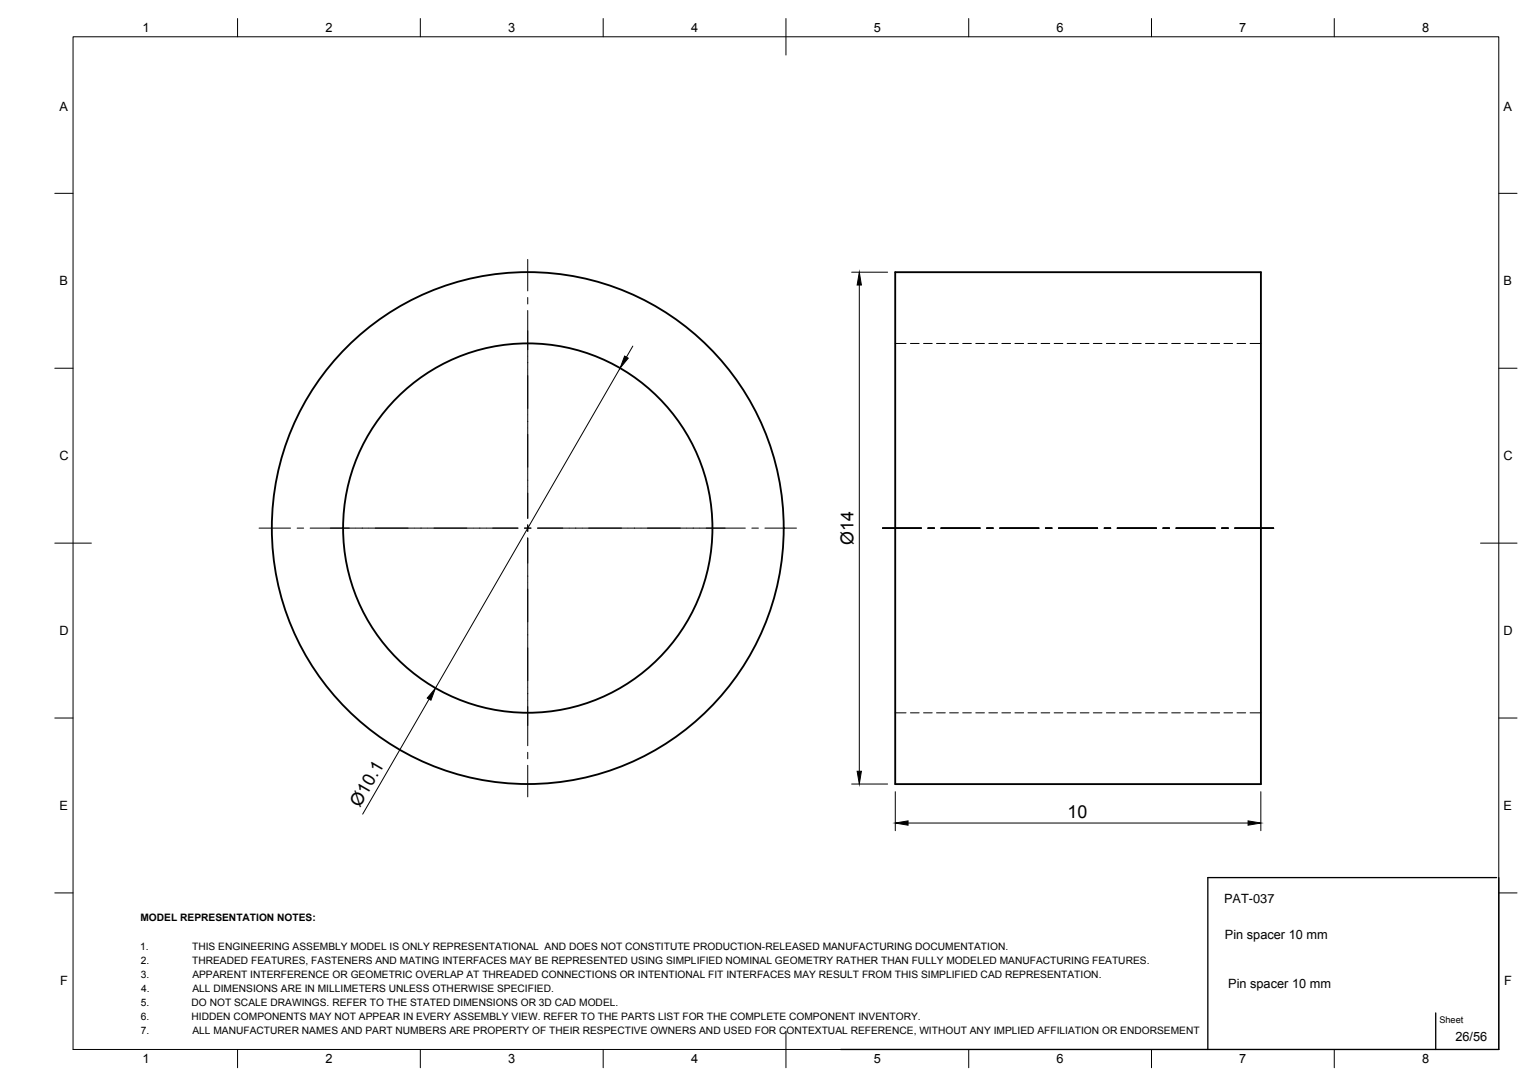
ISO-10303-21;
HEADER;
/* Generated by software containing ST-Developer
 * from STEP Tools, Inc. (www.steptools.com) 
 */

FILE_DESCRIPTION(
/* description */ ('Flywheel Crank-Slider'),
/* implementation_level */ '2;1');

FILE_NAME(
/* name */ 'Pin spacer 10 mm.step',
/* time_stamp */ '2026-10-28T03:23:13-07:00',
/* author */ (''),
/* organization */ (''),
/* preprocessor_version */ 'ST-DEVELOPER v20.2',
/* originating_system */ 'Autodesk Translation Framework v15.17.0.0',
/* authorisation */ '');

FILE_SCHEMA (('AUTOMOTIVE_DESIGN { 1 0 10303 214 3 1 1 }'));
ENDSEC;

DATA;
#10=MECHANICAL_DESIGN_GEOMETRIC_PRESENTATION_REPRESENTATION('',(#696),#17322);
#591=SHAPE_REPRESENTATION_RELATIONSHIP('SRR','None',#17589,#643);
#643=ADVANCED_BREP_SHAPE_REPRESENTATION('',(#753),#17293);
#696=STYLED_ITEM('',(#17931),#753);
#753=MANIFOLD_SOLID_BREP('Body1',#9078);
#924=FACE_BOUND('',#2321,.T.);
#925=FACE_BOUND('',#2323,.T.);
#1205=PLANE('',#10291);
#1206=PLANE('',#10292);
#1644=FACE_OUTER_BOUND('',#2318,.T.);
#1645=FACE_OUTER_BOUND('',#2319,.T.);
#1646=FACE_OUTER_BOUND('',#2320,.T.);
#1647=FACE_OUTER_BOUND('',#2322,.T.);
#2318=EDGE_LOOP('',(#7480,#7481,#7482,#7483));
#2319=EDGE_LOOP('',(#7484,#7485,#7486,#7487));
#2320=EDGE_LOOP('',(#7488));
#2321=EDGE_LOOP('',(#7489));
#2322=EDGE_LOOP('',(#7490));
#2323=EDGE_LOOP('',(#7491));
#3017=LINE('',#15803,#3628);
#3018=LINE('',#15809,#3629);
#3628=VECTOR('',#12435,0.505);
#3629=VECTOR('',#12442,0.7);
#4080=CIRCLE('',#10286,0.505);
#4081=CIRCLE('',#10287,0.505);
#4082=CIRCLE('',#10289,0.7);
#4083=CIRCLE('',#10290,0.7);
#4727=VERTEX_POINT('',#15800);
#4728=VERTEX_POINT('',#15802);
#4729=VERTEX_POINT('',#15806);
#4730=VERTEX_POINT('',#15808);
#5697=EDGE_CURVE('',#4727,#4727,#4080,.T.);
#5698=EDGE_CURVE('',#4727,#4728,#3017,.T.);
#5699=EDGE_CURVE('',#4728,#4728,#4081,.T.);
#5700=EDGE_CURVE('',#4729,#4729,#4082,.T.);
#5701=EDGE_CURVE('',#4729,#4730,#3018,.T.);
#5702=EDGE_CURVE('',#4730,#4730,#4083,.T.);
#7480=ORIENTED_EDGE('',*,*,#5697,.F.);
#7481=ORIENTED_EDGE('',*,*,#5698,.T.);
#7482=ORIENTED_EDGE('',*,*,#5699,.T.);
#7483=ORIENTED_EDGE('',*,*,#5698,.F.);
#7484=ORIENTED_EDGE('',*,*,#5700,.F.);
#7485=ORIENTED_EDGE('',*,*,#5701,.T.);
#7486=ORIENTED_EDGE('',*,*,#5702,.T.);
#7487=ORIENTED_EDGE('',*,*,#5701,.F.);
#7488=ORIENTED_EDGE('',*,*,#5700,.T.);
#7489=ORIENTED_EDGE('',*,*,#5697,.T.);
#7490=ORIENTED_EDGE('',*,*,#5702,.F.);
#7491=ORIENTED_EDGE('',*,*,#5699,.F.);
#8442=CYLINDRICAL_SURFACE('',#10285,0.505);
#8443=CYLINDRICAL_SURFACE('',#10288,0.7);
#8835=ADVANCED_FACE('',(#1644),#8442,.F.);
#8836=ADVANCED_FACE('',(#1645),#8443,.T.);
#8837=ADVANCED_FACE('',(#1646,#924),#1205,.T.);
#8838=ADVANCED_FACE('',(#1647,#925),#1206,.F.);
#9078=CLOSED_SHELL('',(#8835,#8836,#8837,#8838));
#10284=AXIS2_PLACEMENT_3D('',#15798,#12429,#12430);
#10285=AXIS2_PLACEMENT_3D('',#15799,#12431,#12432);
#10286=AXIS2_PLACEMENT_3D('',#15801,#12433,#12434);
#10287=AXIS2_PLACEMENT_3D('',#15804,#12436,#12437);
#10288=AXIS2_PLACEMENT_3D('',#15805,#12438,#12439);
#10289=AXIS2_PLACEMENT_3D('',#15807,#12440,#12441);
#10290=AXIS2_PLACEMENT_3D('',#15810,#12443,#12444);
#10291=AXIS2_PLACEMENT_3D('',#15811,#12445,#12446);
#10292=AXIS2_PLACEMENT_3D('',#15812,#12447,#12448);
#12429=DIRECTION('axis',(0.,0.,1.));
#12430=DIRECTION('refdir',(1.,0.,0.));
#12431=DIRECTION('center_axis',(0.,1.,0.));
#12432=DIRECTION('ref_axis',(1.,0.,0.));
#12433=DIRECTION('center_axis',(0.,-1.,0.));
#12434=DIRECTION('ref_axis',(1.,0.,0.));
#12435=DIRECTION('',(0.,-1.,0.));
#12436=DIRECTION('center_axis',(0.,-1.,0.));
#12437=DIRECTION('ref_axis',(1.,0.,0.));
#12438=DIRECTION('center_axis',(0.,1.,0.));
#12439=DIRECTION('ref_axis',(1.,0.,0.));
#12440=DIRECTION('center_axis',(0.,1.,0.));
#12441=DIRECTION('ref_axis',(1.,0.,0.));
#12442=DIRECTION('',(0.,-1.,0.));
#12443=DIRECTION('center_axis',(0.,1.,0.));
#12444=DIRECTION('ref_axis',(1.,0.,0.));
#12445=DIRECTION('center_axis',(0.,1.,0.));
#12446=DIRECTION('ref_axis',(1.,0.,0.));
#12447=DIRECTION('center_axis',(0.,1.,0.));
#12448=DIRECTION('ref_axis',(1.,0.,0.));
#15798=CARTESIAN_POINT('',(0.,0.,0.));
#15799=CARTESIAN_POINT('Origin',(2.,1.5,10.));
#15800=CARTESIAN_POINT('',(1.495,2.5,10.));
#15801=CARTESIAN_POINT('Origin',(2.,2.5,10.));
#15802=CARTESIAN_POINT('',(1.495,1.5,10.));
#15803=CARTESIAN_POINT('',(1.495,1.5,10.));
#15804=CARTESIAN_POINT('Origin',(2.,1.5,10.));
#15805=CARTESIAN_POINT('Origin',(2.,1.5,10.));
#15806=CARTESIAN_POINT('',(1.3,2.5,10.));
#15807=CARTESIAN_POINT('Origin',(2.,2.5,10.));
#15808=CARTESIAN_POINT('',(1.3,1.5,10.));
#15809=CARTESIAN_POINT('',(1.3,1.5,10.));
#15810=CARTESIAN_POINT('Origin',(2.,1.5,10.));
#15811=CARTESIAN_POINT('Origin',(2.,2.5,10.));
#15812=CARTESIAN_POINT('Origin',(2.,1.5,10.));
#17232=UNCERTAINTY_MEASURE_WITH_UNIT(LENGTH_MEASURE(0.001),#17323,
'DISTANCE_ACCURACY_VALUE',
'Maximum model space distance between geometric entities at asserted c
onnectivities');
#17261=UNCERTAINTY_MEASURE_WITH_UNIT(LENGTH_MEASURE(0.001),#17323,
'DISTANCE_ACCURACY_VALUE',
'Maximum model space distance between geometric entities at asserted c
onnectivities');
#17293=(
GEOMETRIC_REPRESENTATION_CONTEXT(3)
GLOBAL_UNCERTAINTY_ASSIGNED_CONTEXT((#17232))
GLOBAL_UNIT_ASSIGNED_CONTEXT((#17323,#17325,#17326))
REPRESENTATION_CONTEXT('','3D')
);
#17322=(
GEOMETRIC_REPRESENTATION_CONTEXT(3)
GLOBAL_UNCERTAINTY_ASSIGNED_CONTEXT((#17261))
GLOBAL_UNIT_ASSIGNED_CONTEXT((#17323,#17325,#17326))
REPRESENTATION_CONTEXT('','3D')
);
#17323=(
LENGTH_UNIT()
NAMED_UNIT(*)
SI_UNIT(.CENTI.,.METRE.)
);
#17325=(
NAMED_UNIT(*)
PLANE_ANGLE_UNIT()
SI_UNIT($,.RADIAN.)
);
#17326=(
NAMED_UNIT(*)
SI_UNIT($,.STERADIAN.)
SOLID_ANGLE_UNIT()
);
#17358=SHAPE_DEFINITION_REPRESENTATION(#17420,#17589);
#17420=PRODUCT_DEFINITION_SHAPE('',$,#17650);
#17589=SHAPE_REPRESENTATION('',(#10284),#17293);
#17618=PRODUCT_DEFINITION_CONTEXT('part definition',#17800,'design');
#17650=PRODUCT_DEFINITION('Pin spacer 10 mm','Pin spacer 10 mm',#17710,
#17618);
#17710=PRODUCT_DEFINITION_FORMATION('',$,#17833);
#17800=APPLICATION_CONTEXT(
'Core Data for Automotive Mechanical Design Process');
#17801=PRODUCT_CONTEXT('part definition',#17800,'mechanical');
#17833=PRODUCT('Pin spacer 10 mm','Pin spacer 10 mm','Pin spacer 10 mm',
(#17801));
#17925=COLOUR_RGB('Grey',0.48,0.52,0.57);
#17926=FILL_AREA_STYLE_COLOUR('',#17925);
#17927=FILL_AREA_STYLE('',(#17926));
#17928=SURFACE_STYLE_FILL_AREA(#17927);
#17929=SURFACE_SIDE_STYLE('',(#17928));
#17930=SURFACE_STYLE_USAGE(.BOTH.,#17929);
#17931=PRESENTATION_STYLE_ASSIGNMENT((#17930));
ENDSEC;
END-ISO-10303-21;
